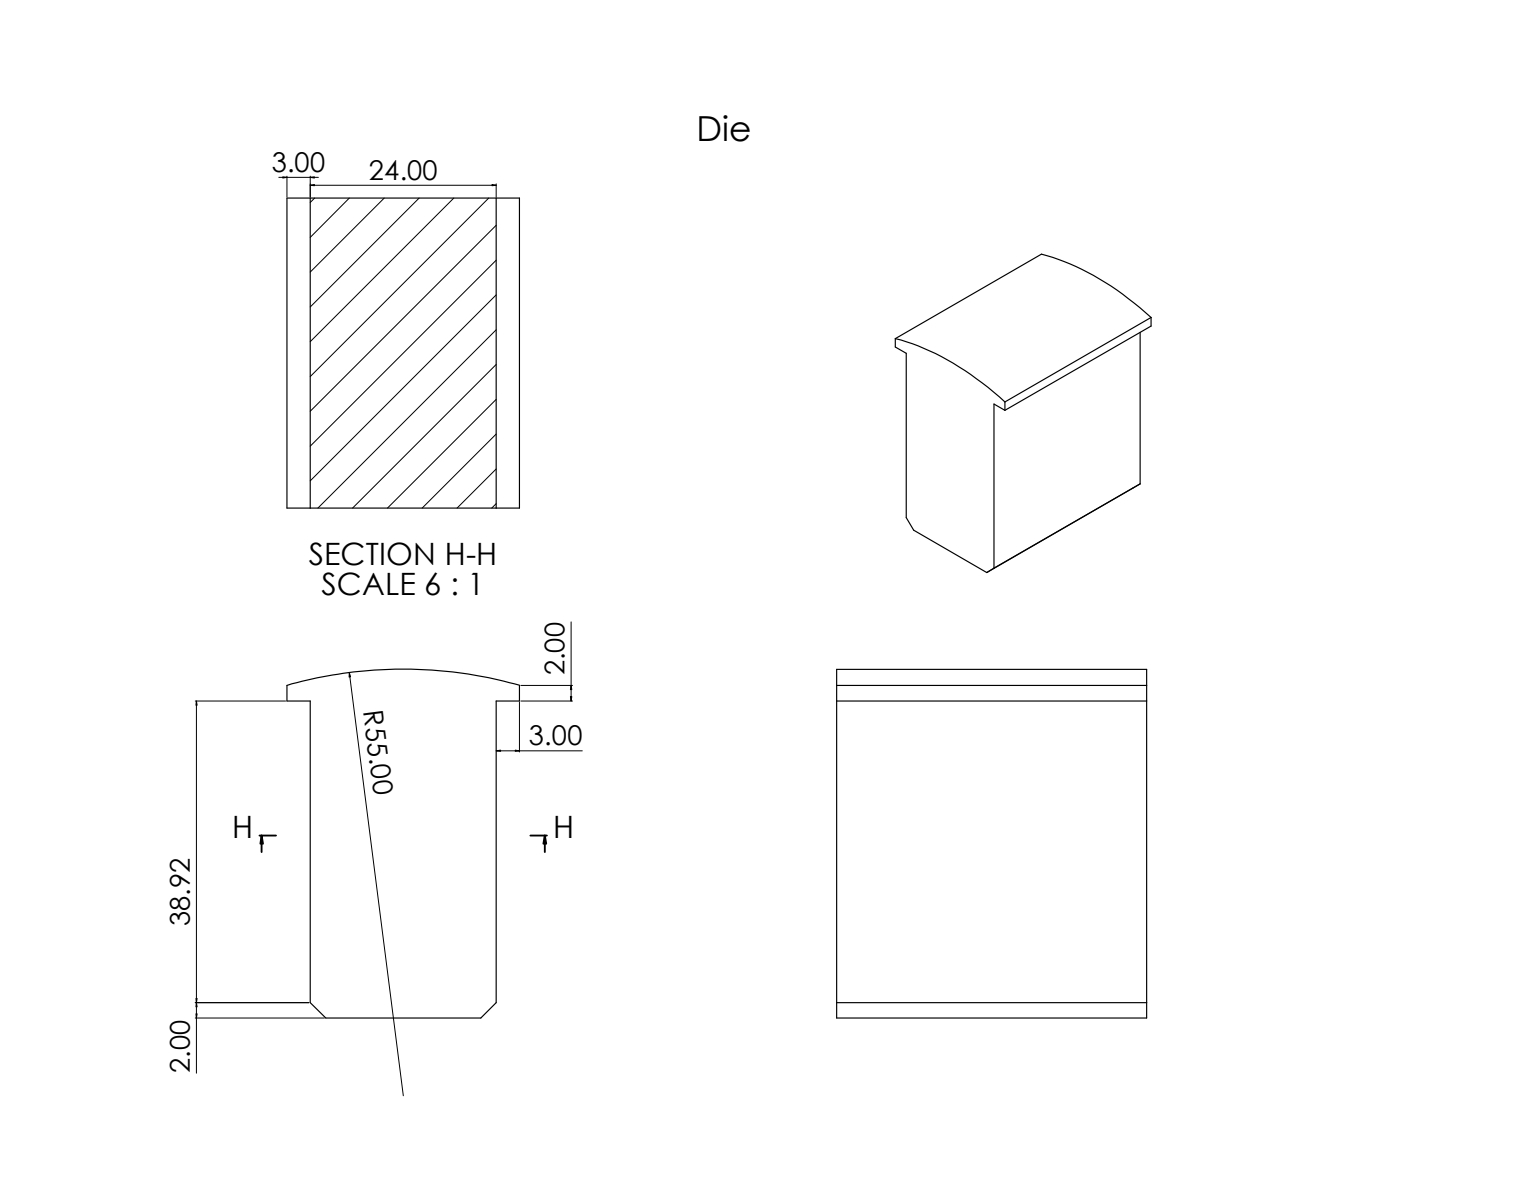
ISO-10303-21;
HEADER;
FILE_DESCRIPTION (('STEP AP214'),
    '1' );
FILE_NAME ('Die.step',
    '2026-10-25T19:19:31',
    ( '' ),
    ( '' ),
    'SwSTEP 2.0',
    'SolidWorks 2025',
    '' );
FILE_SCHEMA (( 'AUTOMOTIVE_DESIGN' ));
ENDSEC;

DATA;
#6=LINE ( 'NONE', #939, #4428 ) ;
#19=( NAMED_UNIT ( * ) SI_UNIT ( $, .STERADIAN. ) SOLID_ANGLE_UNIT ( ) );
#35=DIRECTION ( 'NONE',  ( 0.000000000000000000, -1.000000000000000000, 0.000000000000000000 ) ) ;
#40=APPLICATION_CONTEXT ( 'automotive_design' ) ;
#41=EDGE_CURVE ( 'NONE', #1178, #2811, #1439, .T. ) ;
#54=ORIENTED_EDGE ( 'NONE', *, *, #4887, .F. ) ;
#73=AXIS2_PLACEMENT_3D ( 'NONE', #3304, #3763, #5645 ) ;
#85=ORIENTED_EDGE ( 'NONE', *, *, #1081, .T. ) ;
#90=EDGE_CURVE ( 'NONE', #1861, #5383, #5968, .T. ) ;
#100=VECTOR ( 'NONE', #4962, 1000.000000000000000 ) ;
#127=EDGE_CURVE ( 'NONE', #4172, #3364, #4015, .T. ) ;
#185=EDGE_LOOP ( 'NONE', ( #533, #4724, #4763, #1601 ) ) ;
#202=AXIS2_PLACEMENT_3D ( 'NONE', #584, #4355, #522 ) ;
#232=ORIENTED_EDGE ( 'NONE', *, *, #1098, .F. ) ;
#233=FACE_OUTER_BOUND ( 'NONE', #1137, .T. ) ;
#242=ORIENTED_EDGE ( 'NONE', *, *, #2892, .F. ) ;
#249=MANIFOLD_SOLID_BREP ( 'Boss-Extrude4', #1653 ) ;
#255=LINE ( 'NONE', #729, #5225 ) ;
#274=DIRECTION ( 'NONE',  ( 0.000000000000000000, -1.000000000000000000, 0.000000000000000000 ) ) ;
#278=EDGE_LOOP ( 'NONE', ( #2591, #3538, #5453, #1395 ) ) ;
#289=DIRECTION ( 'NONE',  ( -0.000000000000000000, -0.000000000000000000, -1.000000000000000000 ) ) ;
#292=ADVANCED_FACE ( 'NONE', ( #988 ), #5742, .F. ) ;
#307=LINE ( 'NONE', #5608, #5057 ) ;
#321=DIRECTION ( 'NONE',  ( 1.000000000000000000, 8.673617379884026597E-16, -0.000000000000000000 ) ) ;
#329=PLANE ( 'NONE',  #2861 ) ;
#338=DIRECTION ( 'NONE',  ( -0.000000000000000000, -0.000000000000000000, -1.000000000000000000 ) ) ;
#350=EDGE_CURVE ( 'NONE', #4063, #382, #1866, .T. ) ;
#354=VERTEX_POINT ( 'NONE', #4776 ) ;
#382=VERTEX_POINT ( 'NONE', #5209 ) ;
#416=CARTESIAN_POINT ( 'NONE',  ( -15.00000000000000178, 52.91502622129182498, -20.00000000000000000 ) ) ;
#440=ORIENTED_EDGE ( 'NONE', *, *, #2522, .F. ) ;
#444=LINE ( 'NONE', #1490, #3945 ) ;
#451=CARTESIAN_POINT ( 'NONE',  ( -10.00000000000000178, 10.00000000000000178, -20.00000000000000000 ) ) ;
#475=AXIS2_PLACEMENT_3D ( 'NONE', #1088, #2025, #3550 ) ;
#489=ORIENTED_EDGE ( 'NONE', *, *, #127, .F. ) ;
#516=ORIENTED_EDGE ( 'NONE', *, *, #2045, .F. ) ;
#521=EDGE_CURVE ( 'NONE', #4734, #5727, #5427, .T. ) ;
#522=DIRECTION ( 'NONE',  ( -1.000000000000000000, 0.000000000000000000, 0.000000000000000000 ) ) ;
#533=ORIENTED_EDGE ( 'NONE', *, *, #4248, .T. ) ;
#546=ORIENTED_EDGE ( 'NONE', *, *, #4887, .T. ) ;
#584=CARTESIAN_POINT ( 'NONE',  ( 0.000000000000000000, 0.000000000000000000, 20.00000000000000000 ) ) ;
#636=ORIENTED_EDGE ( 'NONE', *, *, #827, .T. ) ;
#686=PLANE ( 'NONE',  #475 ) ;
#687=VECTOR ( 'NONE', #1691, 1000.000000000000000 ) ;
#707=VECTOR ( 'NONE', #2728, 1000.000000000000000 ) ;
#729=CARTESIAN_POINT ( 'NONE',  ( 9.999999999999998224, 9.999999999999998224, 20.00000000000000000 ) ) ;
#763=AXIS2_PLACEMENT_3D ( 'NONE', #4089, #6004, #1717 ) ;
#772=DIRECTION ( 'NONE',  ( -0.000000000000000000, 0.000000000000000000, 1.000000000000000000 ) ) ;
#773=LINE ( 'NONE', #3989, #1060 ) ;
#789=PLANE ( 'NONE',  #3246 ) ;
#793=EDGE_CURVE ( 'NONE', #354, #5786, #5696, .T. ) ;
#803=( GEOMETRIC_REPRESENTATION_CONTEXT ( 3 ) GLOBAL_UNCERTAINTY_ASSIGNED_CONTEXT ( ( #3805 ) ) GLOBAL_UNIT_ASSIGNED_CONTEXT ( ( #5845, #5678, #19 ) ) REPRESENTATION_CONTEXT ( 'NONE', 'WORKASPACE' ) );
#821=DIRECTION ( 'NONE',  ( 1.000000000000000000, -5.329070518200750605E-15, 0.000000000000000000 ) ) ;
#827=EDGE_CURVE ( 'NONE', #4272, #1861, #444, .T. ) ;
#870=VECTOR ( 'NONE', #3518, 1000.000000000000000 ) ;
#875=( GEOMETRIC_REPRESENTATION_CONTEXT ( 3 ) GLOBAL_UNCERTAINTY_ASSIGNED_CONTEXT ( ( #4308 ) ) GLOBAL_UNIT_ASSIGNED_CONTEXT ( ( #2245, #2215, #3729 ) ) REPRESENTATION_CONTEXT ( 'NONE', 'WORKASPACE' ) );
#898=SHAPE_REPRESENTATION_RELATIONSHIP ( 'NONE' , 'NONE' ,  #2176, #5744 ) ;
#930=LINE ( 'NONE', #958, #6029 ) ;
#939=CARTESIAN_POINT ( 'NONE',  ( -15.00000000000000178, 52.91502622129182498, 20.00000000000000000 ) ) ;
#945=VERTEX_POINT ( 'NONE', #1038 ) ;
#949=DIRECTION ( 'NONE',  ( -0.000000000000000000, -0.000000000000000000, -1.000000000000000000 ) ) ;
#958=CARTESIAN_POINT ( 'NONE',  ( 15.00000000000000178, 52.91502622129182498, 20.00000000000000000 ) ) ;
#970=PRODUCT ( 'Die', 'Die', '', ( #2146 ) ) ;
#988=FACE_OUTER_BOUND ( 'NONE', #1209, .T. ) ;
#992=VECTOR ( 'NONE', #1588, 1000.000000000000000 ) ;
#1022=DIRECTION ( 'NONE',  ( 1.000000000000000000, 0.000000000000000000, -0.000000000000000000 ) ) ;
#1038=CARTESIAN_POINT ( 'NONE',  ( -12.00000000000000000, 50.91502622129181788, 20.00000000000000000 ) ) ;
#1049=DIRECTION ( 'NONE',  ( -0.7071067811865469066, -0.7071067811865482389, 0.000000000000000000 ) ) ;
#1060=VECTOR ( 'NONE', #5434, 1000.000000000000000 ) ;
#1078=CARTESIAN_POINT ( 'NONE',  ( 12.00000000000000000, 50.91502622129181788, 20.00000000000000000 ) ) ;
#1081=EDGE_CURVE ( 'NONE', #1820, #382, #1825, .T. ) ;
#1088=CARTESIAN_POINT ( 'NONE',  ( 0.000000000000000000, 50.91502622129181788, 20.00000000000000000 ) ) ;
#1098=EDGE_CURVE ( 'NONE', #945, #1834, #307, .T. ) ;
#1110=DIRECTION ( 'NONE',  ( 0.000000000000000000, 1.000000000000000000, 0.000000000000000000 ) ) ;
#1122=ADVANCED_FACE ( 'NONE', ( #2775 ), #6053, .T. ) ;
#1131=ORIENTED_EDGE ( 'NONE', *, *, #5292, .T. ) ;
#1137=EDGE_LOOP ( 'NONE', ( #4292, #4354, #2571, #1131 ) ) ;
#1178=VERTEX_POINT ( 'NONE', #5278 ) ;
#1184=DIRECTION ( 'NONE',  ( -0.000000000000000000, 0.000000000000000000, 1.000000000000000000 ) ) ;
#1209=EDGE_LOOP ( 'NONE', ( #1696, #440, #232, #3423 ) ) ;
#1227=DIRECTION ( 'NONE',  ( 0.000000000000000000, -1.000000000000000000, 0.000000000000000000 ) ) ;
#1237=DIRECTION ( 'NONE',  ( -1.000000000000000000, 0.000000000000000000, 0.000000000000000000 ) ) ;
#1239=ORIENTED_EDGE ( 'NONE', *, *, #827, .F. ) ;
#1283=PLANE ( 'NONE',  #3222 ) ;
#1302=VERTEX_POINT ( 'NONE', #451 ) ;
#1335=VECTOR ( 'NONE', #338, 1000.000000000000000 ) ;
#1348=CIRCLE ( 'NONE', #2556, 55.00000000000001421 ) ;
#1387=PRODUCT_DEFINITION ( 'UNKNOWN', '', #4631, #2453 ) ;
#1392=DIRECTION ( 'NONE',  ( -0.000000000000000000, -0.000000000000000000, -1.000000000000000000 ) ) ;
#1395=ORIENTED_EDGE ( 'NONE', *, *, #3668, .T. ) ;
#1399=EDGE_CURVE ( 'NONE', #1672, #3029, #3458, .T. ) ;
#1405=CARTESIAN_POINT ( 'NONE',  ( 8.586443133426902668E-15, -8.586443133426886890E-15, 20.00000000000000000 ) ) ;
#1411=DIRECTION ( 'NONE',  ( -8.673617379884026597E-16, -1.000000000000000000, 0.000000000000000000 ) ) ;
#1424=CARTESIAN_POINT ( 'NONE',  ( -12.00000000000000000, 50.91502622129181788, -20.00000000000000000 ) ) ;
#1426=CARTESIAN_POINT ( 'NONE',  ( -11.99999999999999645, 12.00000000000000355, -20.00000000000000000 ) ) ;
#1439=LINE ( 'NONE', #2975, #4855 ) ;
#1490=CARTESIAN_POINT ( 'NONE',  ( 12.00000000000000000, 0.000000000000000000, -20.00000000000000000 ) ) ;
#1509=ORIENTED_EDGE ( 'NONE', *, *, #2047, .F. ) ;
#1525=DIRECTION ( 'NONE',  ( -0.000000000000000000, 0.000000000000000000, -1.000000000000000000 ) ) ;
#1530=ORIENTED_EDGE ( 'NONE', *, *, #2087, .T. ) ;
#1541=VECTOR ( 'NONE', #6048, 1000.000000000000000 ) ;
#1565=ADVANCED_FACE ( 'NONE', ( #5516 ), #329, .T. ) ;
#1571=VECTOR ( 'NONE', #5524, 1000.000000000000000 ) ;
#1583=FACE_OUTER_BOUND ( 'NONE', #278, .T. ) ;
#1588=DIRECTION ( 'NONE',  ( 8.673617379884026597E-16, -1.000000000000000000, 0.000000000000000000 ) ) ;
#1597=ORIENTED_EDGE ( 'NONE', *, *, #5103, .F. ) ;
#1601=ORIENTED_EDGE ( 'NONE', *, *, #2522, .T. ) ;
#1605=DIRECTION ( 'NONE',  ( 0.000000000000000000, -0.000000000000000000, -1.000000000000000000 ) ) ;
#1629=EDGE_CURVE ( 'NONE', #354, #1672, #6, .T. ) ;
#1651=CARTESIAN_POINT ( 'NONE',  ( -12.00000000000000000, 0.000000000000000000, -20.00000000000000000 ) ) ;
#1653=CLOSED_SHELL ( 'NONE', ( #3387, #2095, #2312, #292, #4074, #4285, #1565, #5408, #3225, #5043, #1122, #5390 ) ) ;
#1665=CARTESIAN_POINT ( 'NONE',  ( 9.999999999999998224, 9.999999999999998224, -20.00000000000000000 ) ) ;
#1672=VERTEX_POINT ( 'NONE', #416 ) ;
#1675=CARTESIAN_POINT ( 'NONE',  ( 8.586443133426902668E-15, -8.586443133426886890E-15, 20.00000000000000000 ) ) ;
#1691=DIRECTION ( 'NONE',  ( 0.000000000000000000, -1.000000000000000000, 0.000000000000000000 ) ) ;
#1692=FACE_OUTER_BOUND ( 'NONE', #4176, .T. ) ;
#1695=LINE ( 'NONE', #3172, #5157 ) ;
#1696=ORIENTED_EDGE ( 'NONE', *, *, #127, .T. ) ;
#1715=LINE ( 'NONE', #2497, #3224 ) ;
#1717=DIRECTION ( 'NONE',  ( -0.000000000000000000, 0.000000000000000000, -1.000000000000000000 ) ) ;
#1740=DIRECTION ( 'NONE',  ( 8.673617379884026597E-16, 1.000000000000000000, 0.000000000000000000 ) ) ;
#1758=DIRECTION ( 'NONE',  ( -0.000000000000000000, -0.000000000000000000, -1.000000000000000000 ) ) ;
#1820=VERTEX_POINT ( 'NONE', #3412 ) ;
#1825=LINE ( 'NONE', #4166, #1571 ) ;
#1834=VERTEX_POINT ( 'NONE', #4412 ) ;
#1861=VERTEX_POINT ( 'NONE', #3450 ) ;
#1866=LINE ( 'NONE', #1405, #5761 ) ;
#1945=CARTESIAN_POINT ( 'NONE',  ( -15.00000000000000000, 50.91502622129181788, 20.00000000000000000 ) ) ;
#1959=ORIENTED_EDGE ( 'NONE', *, *, #521, .T. ) ;
#1963=DIRECTION ( 'NONE',  ( -0.000000000000000000, -0.000000000000000000, -1.000000000000000000 ) ) ;
#1984=EDGE_CURVE ( 'NONE', #1302, #5383, #2197, .T. ) ;
#2025=DIRECTION ( 'NONE',  ( 0.000000000000000000, -1.000000000000000000, 0.000000000000000000 ) ) ;
#2032=CARTESIAN_POINT ( 'NONE',  ( -1.594625153350711036E-14, -1.594625153350706303E-14, 20.00000000000000000 ) ) ;
#2045=EDGE_CURVE ( 'NONE', #354, #4734, #1348, .T. ) ;
#2047=EDGE_CURVE ( 'NONE', #2811, #4272, #2698, .T. ) ;
#2087=EDGE_CURVE ( 'NONE', #3324, #4063, #3707, .T. ) ;
#2091=DIRECTION ( 'NONE',  ( -0.7071067811865469066, -0.7071067811865482389, 0.000000000000000000 ) ) ;
#2094=LINE ( 'NONE', #2032, #2125 ) ;
#2095=ADVANCED_FACE ( 'NONE', ( #3592 ), #789, .F. ) ;
#2110=SHAPE_DEFINITION_REPRESENTATION ( #3775, #2176 ) ;
#2125=VECTOR ( 'NONE', #5971, 1000.000000000000000 ) ;
#2146=PRODUCT_CONTEXT ( 'NONE', #40, 'mechanical' ) ;
#2156=ORIENTED_EDGE ( 'NONE', *, *, #5112, .T. ) ;
#2166=DIRECTION ( 'NONE',  ( 0.000000000000000000, -0.000000000000000000, -1.000000000000000000 ) ) ;
#2176=SHAPE_REPRESENTATION ( 'Die', ( #73 ), #875 ) ;
#2197=LINE ( 'NONE', #4625, #4943 ) ;
#2198=FACE_OUTER_BOUND ( 'NONE', #4368, .T. ) ;
#2215=( NAMED_UNIT ( * ) PLANE_ANGLE_UNIT ( ) SI_UNIT ( $, .RADIAN. ) );
#2245=( LENGTH_UNIT ( ) NAMED_UNIT ( * ) SI_UNIT ( .MILLI., .METRE. ) );
#2312=ADVANCED_FACE ( 'NONE', ( #233 ), #3139, .F. ) ;
#2313=ORIENTED_EDGE ( 'NONE', *, *, #5292, .F. ) ;
#2405=CARTESIAN_POINT ( 'NONE',  ( 15.00000000000000000, 50.91502622129181788, 20.00000000000000000 ) ) ;
#2453=PRODUCT_DEFINITION_CONTEXT ( 'detailed design', #2895, 'design' ) ;
#2463=CYLINDRICAL_SURFACE ( 'NONE', #202, 55.00000000000001421 ) ;
#2497=CARTESIAN_POINT ( 'NONE',  ( -1.594625153350711036E-14, -1.594625153350706303E-14, -20.00000000000000000 ) ) ;
#2522=EDGE_CURVE ( 'NONE', #1834, #3364, #3629, .T. ) ;
#2530=ORIENTED_EDGE ( 'NONE', *, *, #793, .T. ) ;
#2532=CARTESIAN_POINT ( 'NONE',  ( 14.99999999999995559, -1.301042606982600272E-14, 20.00000000000000000 ) ) ;
#2554=ORIENTED_EDGE ( 'NONE', *, *, #5378, .T. ) ;
#2556=AXIS2_PLACEMENT_3D ( 'NONE', #5101, #2166, #821 ) ;
#2559=DIRECTION ( 'NONE',  ( -0.000000000000000000, -0.000000000000000000, -1.000000000000000000 ) ) ;
#2571=ORIENTED_EDGE ( 'NONE', *, *, #3951, .F. ) ;
#2578=ORIENTED_EDGE ( 'NONE', *, *, #350, .F. ) ;
#2589=ORIENTED_EDGE ( 'NONE', *, *, #4893, .T. ) ;
#2591=ORIENTED_EDGE ( 'NONE', *, *, #1984, .T. ) ;
#2601=LINE ( 'NONE', #3962, #870 ) ;
#2618=EDGE_LOOP ( 'NONE', ( #516, #2530, #3475, #3498, #3096, #85, #2578, #3782, #54, #4075 ) ) ;
#2659=EDGE_LOOP ( 'NONE', ( #4184, #2313, #4641, #4438 ) ) ;
#2671=CARTESIAN_POINT ( 'NONE',  ( 0.000000000000000000, 0.000000000000000000, -20.00000000000000000 ) ) ;
#2686=LINE ( 'NONE', #4585, #1335 ) ;
#2698=LINE ( 'NONE', #4594, #5544 ) ;
#2699=PLANE ( 'NONE',  #763 ) ;
#2728=DIRECTION ( 'NONE',  ( -0.000000000000000000, -0.000000000000000000, -1.000000000000000000 ) ) ;
#2754=ORIENTED_EDGE ( 'NONE', *, *, #1984, .F. ) ;
#2775=FACE_OUTER_BOUND ( 'NONE', #2618, .T. ) ;
#2797=CARTESIAN_POINT ( 'NONE',  ( 12.00000000000000000, 12.00000000000000355, 20.00000000000000000 ) ) ;
#2811=VERTEX_POINT ( 'NONE', #6137 ) ;
#2814=ORIENTED_EDGE ( 'NONE', *, *, #5103, .T. ) ;
#2861=AXIS2_PLACEMENT_3D ( 'NONE', #1675, #3111, #5602 ) ;
#2890=DIRECTION ( 'NONE',  ( -0.7071067811865464625, 0.7071067811865486830, 0.000000000000000000 ) ) ;
#2892=EDGE_CURVE ( 'NONE', #3029, #4172, #1695, .T. ) ;
#2895=APPLICATION_CONTEXT ( 'automotive_design' ) ;
#2949=AXIS2_PLACEMENT_3D ( 'NONE', #3544, #4506, #4541 ) ;
#2975=CARTESIAN_POINT ( 'NONE',  ( 14.99999999999995559, -1.301042606982600272E-14, -20.00000000000000000 ) ) ;
#2992=EDGE_LOOP ( 'NONE', ( #1597, #5836, #5687, #3359 ) ) ;
#3029=VERTEX_POINT ( 'NONE', #5195 ) ;
#3076=DIRECTION ( 'NONE',  ( 1.000000000000000000, 0.000000000000000000, 0.000000000000000000 ) ) ;
#3093=CARTESIAN_POINT ( 'NONE',  ( 8.586443133426902668E-15, -8.586443133426886890E-15, -20.00000000000000000 ) ) ;
#3096=ORIENTED_EDGE ( 'NONE', *, *, #4794, .T. ) ;
#3111=DIRECTION ( 'NONE',  ( 0.7071067811865482389, -0.7071067811865469066, 0.000000000000000000 ) ) ;
#3115=CARTESIAN_POINT ( 'NONE',  ( 12.00000000000000000, 50.91502622129181788, 20.00000000000000000 ) ) ;
#3139=PLANE ( 'NONE',  #2949 ) ;
#3140=ORIENTED_EDGE ( 'NONE', *, *, #4248, .F. ) ;
#3156=ORIENTED_EDGE ( 'NONE', *, *, #5799, .F. ) ;
#3158=STYLED_ITEM('',(#6170),#249);
#3172=CARTESIAN_POINT ( 'NONE',  ( -0.000000000000000000, 50.91502622129181788, -20.00000000000000000 ) ) ;
#3201=ORIENTED_EDGE ( 'NONE', *, *, #350, .T. ) ;
#3222=AXIS2_PLACEMENT_3D ( 'NONE', #5091, #5060, #1740 ) ;
#3224=VECTOR ( 'NONE', #5298, 1000.000000000000000 ) ;
#3225=ADVANCED_FACE ( 'NONE', ( #5963 ), #686, .T. ) ;
#3246=AXIS2_PLACEMENT_3D ( 'NONE', #4088, #321, #6003 ) ;
#3291=ORIENTED_EDGE ( 'NONE', *, *, #2047, .T. ) ;
#3304=CARTESIAN_POINT ( 'NONE',  ( 0.000000000000000000, 0.000000000000000000, 0.000000000000000000 ) ) ;
#3324=VERTEX_POINT ( 'NONE', #3115 ) ;
#3331=LINE ( 'NONE', #2405, #5825 ) ;
#3359=ORIENTED_EDGE ( 'NONE', *, *, #5799, .T. ) ;
#3364=VERTEX_POINT ( 'NONE', #1426 ) ;
#3367=CARTESIAN_POINT ( 'NONE',  ( -12.00000000000000000, 0.000000000000000000, 20.00000000000000000 ) ) ;
#3387=ADVANCED_FACE ( 'NONE', ( #4289 ), #2463, .T. ) ;
#3412=CARTESIAN_POINT ( 'NONE',  ( -10.00000000000000178, 10.00000000000000178, 20.00000000000000000 ) ) ;
#3423=ORIENTED_EDGE ( 'NONE', *, *, #5072, .T. ) ;
#3450=CARTESIAN_POINT ( 'NONE',  ( 12.00000000000000000, 12.00000000000000355, -20.00000000000000000 ) ) ;
#3458=LINE ( 'NONE', #3917, #992 ) ;
#3475=ORIENTED_EDGE ( 'NONE', *, *, #3951, .T. ) ;
#3481=DIRECTION ( 'NONE',  ( 0.000000000000000000, -0.000000000000000000, 1.000000000000000000 ) ) ;
#3498=ORIENTED_EDGE ( 'NONE', *, *, #1098, .T. ) ;
#3500=EDGE_CURVE ( 'NONE', #3324, #4272, #4898, .T. ) ;
#3518=DIRECTION ( 'NONE',  ( -1.000000000000000000, 0.000000000000000000, 0.000000000000000000 ) ) ;
#3538=ORIENTED_EDGE ( 'NONE', *, *, #5378, .F. ) ;
#3544=CARTESIAN_POINT ( 'NONE',  ( 0.000000000000000000, 50.91502622129181788, 20.00000000000000000 ) ) ;
#3550=DIRECTION ( 'NONE',  ( 0.000000000000000000, -0.000000000000000000, -1.000000000000000000 ) ) ;
#3552=VECTOR ( 'NONE', #4258, 1000.000000000000000 ) ;
#3563=VECTOR ( 'NONE', #1963, 1000.000000000000000 ) ;
#3592=FACE_OUTER_BOUND ( 'NONE', #2659, .T. ) ;
#3593=PLANE ( 'NONE',  #4824 ) ;
#3595=DIRECTION ( 'NONE',  ( 1.000000000000000000, 0.000000000000000000, 0.000000000000000000 ) ) ;
#3611=ORIENTED_EDGE ( 'NONE', *, *, #1399, .F. ) ;
#3619=AXIS2_PLACEMENT_3D ( 'NONE', #4316, #6102, #2890 ) ;
#3629=LINE ( 'NONE', #5547, #707 ) ;
#3668=EDGE_CURVE ( 'NONE', #1820, #1302, #6111, .T. ) ;
#3707=LINE ( 'NONE', #5978, #687 ) ;
#3709=AXIS2_PLACEMENT_3D ( 'NONE', #4295, #1605, #4228 ) ;
#3729=( NAMED_UNIT ( * ) SI_UNIT ( $, .STERADIAN. ) SOLID_ANGLE_UNIT ( ) );
#3735=EDGE_LOOP ( 'NONE', ( #4808, #4256, #3201, #2554 ) ) ;
#3760=CARTESIAN_POINT ( 'NONE',  ( -15.00000000000000000, 50.91502622129181788, 20.00000000000000000 ) ) ;
#3763=DIRECTION ( 'NONE',  ( 0.000000000000000000, 0.000000000000000000, 1.000000000000000000 ) ) ;
#3775=PRODUCT_DEFINITION_SHAPE ( 'NONE', 'NONE',  #1387 ) ;
#3782=ORIENTED_EDGE ( 'NONE', *, *, #2087, .F. ) ;
#3805=UNCERTAINTY_MEASURE_WITH_UNIT (LENGTH_MEASURE( 1.000000000000000082E-05 ), #5845, 'distance_accuracy_value', 'NONE');
#3808=EDGE_LOOP ( 'NONE', ( #1509, #5655, #546, #5484 ) ) ;
#3849=FACE_OUTER_BOUND ( 'NONE', #185, .T. ) ;
#3901=ORIENTED_EDGE ( 'NONE', *, *, #41, .F. ) ;
#3917=CARTESIAN_POINT ( 'NONE',  ( -14.99999999999995559, -1.301042606982600272E-14, -20.00000000000000000 ) ) ;
#3944=CARTESIAN_POINT ( 'NONE',  ( 12.00000000000000000, 50.91502622129181788, -20.00000000000000000 ) ) ;
#3945=VECTOR ( 'NONE', #35, 1000.000000000000000 ) ;
#3951=EDGE_CURVE ( 'NONE', #5786, #945, #4134, .T. ) ;
#3962=CARTESIAN_POINT ( 'NONE',  ( 0.000000000000000000, 50.91502622129181788, 20.00000000000000000 ) ) ;
#3977=ORIENTED_EDGE ( 'NONE', *, *, #90, .T. ) ;
#3989=CARTESIAN_POINT ( 'NONE',  ( 12.00000000000000000, 12.00000000000000355, 20.00000000000000000 ) ) ;
#4015=LINE ( 'NONE', #1651, #4234 ) ;
#4063=VERTEX_POINT ( 'NONE', #2797 ) ;
#4074=ADVANCED_FACE ( 'NONE', ( #3849 ), #4695, .F. ) ;
#4075=ORIENTED_EDGE ( 'NONE', *, *, #521, .F. ) ;
#4088=CARTESIAN_POINT ( 'NONE',  ( -14.99999999999995559, -1.301042606982600272E-14, 20.00000000000000000 ) ) ;
#4089=CARTESIAN_POINT ( 'NONE',  ( 12.00000000000000000, 0.000000000000000000, 20.00000000000000000 ) ) ;
#4134=LINE ( 'NONE', #4162, #1541 ) ;
#4162=CARTESIAN_POINT ( 'NONE',  ( 0.000000000000000000, 50.91502622129181788, 20.00000000000000000 ) ) ;
#4166=CARTESIAN_POINT ( 'NONE',  ( 0.000000000000000000, 9.999999999999998224, 20.00000000000000000 ) ) ;
#4172=VERTEX_POINT ( 'NONE', #1424 ) ;
#4176=EDGE_LOOP ( 'NONE', ( #2814, #5535, #3291, #636, #3977, #2754, #3140, #489, #242, #3611 ) ) ;
#4184=ORIENTED_EDGE ( 'NONE', *, *, #1399, .T. ) ;
#4228=DIRECTION ( 'NONE',  ( 1.000000000000000000, -5.329070518200750605E-15, 0.000000000000000000 ) ) ;
#4234=VECTOR ( 'NONE', #274, 1000.000000000000000 ) ;
#4238=DIRECTION ( 'NONE',  ( -0.000000000000000000, -0.000000000000000000, -1.000000000000000000 ) ) ;
#4248=EDGE_CURVE ( 'NONE', #3364, #1302, #1715, .T. ) ;
#4256=ORIENTED_EDGE ( 'NONE', *, *, #4893, .F. ) ;
#4258=DIRECTION ( 'NONE',  ( 8.673617379884026597E-16, -1.000000000000000000, 0.000000000000000000 ) ) ;
#4272=VERTEX_POINT ( 'NONE', #3944 ) ;
#4285=ADVANCED_FACE ( 'NONE', ( #1583 ), #5829, .F. ) ;
#4289=FACE_OUTER_BOUND ( 'NONE', #2992, .T. ) ;
#4292=ORIENTED_EDGE ( 'NONE', *, *, #2892, .T. ) ;
#4295=CARTESIAN_POINT ( 'NONE',  ( 0.000000000000000000, 0.000000000000000000, -20.00000000000000000 ) ) ;
#4308=UNCERTAINTY_MEASURE_WITH_UNIT (LENGTH_MEASURE( 1.000000000000000082E-05 ), #2245, 'distance_accuracy_value', 'NONE');
#4315=CIRCLE ( 'NONE', #3709, 55.00000000000001421 ) ;
#4316=CARTESIAN_POINT ( 'NONE',  ( -1.594625153350711036E-14, -1.594625153350706303E-14, 20.00000000000000000 ) ) ;
#4354=ORIENTED_EDGE ( 'NONE', *, *, #5072, .F. ) ;
#4355=DIRECTION ( 'NONE',  ( -0.000000000000000000, -0.000000000000000000, -1.000000000000000000 ) ) ;
#4368=EDGE_LOOP ( 'NONE', ( #1239, #5607, #1530, #2589 ) ) ;
#4412=CARTESIAN_POINT ( 'NONE',  ( -11.99999999999999645, 12.00000000000000355, 20.00000000000000000 ) ) ;
#4428=VECTOR ( 'NONE', #1392, 1000.000000000000000 ) ;
#4438=ORIENTED_EDGE ( 'NONE', *, *, #1629, .T. ) ;
#4506=DIRECTION ( 'NONE',  ( 0.000000000000000000, 1.000000000000000000, 0.000000000000000000 ) ) ;
#4541=DIRECTION ( 'NONE',  ( 0.000000000000000000, -0.000000000000000000, 1.000000000000000000 ) ) ;
#4551=DIRECTION ( 'NONE',  ( 1.000000000000000000, 0.000000000000000000, 0.000000000000000000 ) ) ;
#4559=AXIS2_PLACEMENT_3D ( 'NONE', #3367, #1022, #1525 ) ;
#4565=CARTESIAN_POINT ( 'NONE',  ( 15.00000000000000000, 50.91502622129181788, 20.00000000000000000 ) ) ;
#4585=CARTESIAN_POINT ( 'NONE',  ( -12.00000000000000000, 50.91502622129181788, 20.00000000000000000 ) ) ;
#4594=CARTESIAN_POINT ( 'NONE',  ( 0.000000000000000000, 50.91502622129181788, -20.00000000000000000 ) ) ;
#4625=CARTESIAN_POINT ( 'NONE',  ( -0.000000000000000000, 9.999999999999998224, -20.00000000000000000 ) ) ;
#4631=PRODUCT_DEFINITION_FORMATION_WITH_SPECIFIED_SOURCE ( 'ANY', '', #970, .NOT_KNOWN. ) ;
#4641=ORIENTED_EDGE ( 'NONE', *, *, #793, .F. ) ;
#4658=DIRECTION ( 'NONE',  ( 1.000000000000000000, 0.000000000000000000, 0.000000000000000000 ) ) ;
#4695=PLANE ( 'NONE',  #3619 ) ;
#4724=ORIENTED_EDGE ( 'NONE', *, *, #3668, .F. ) ;
#4726=AXIS2_PLACEMENT_3D ( 'NONE', #5328, #1110, #3481 ) ;
#4734=VERTEX_POINT ( 'NONE', #5908 ) ;
#4763=ORIENTED_EDGE ( 'NONE', *, *, #4794, .F. ) ;
#4776=CARTESIAN_POINT ( 'NONE',  ( -15.00000000000000178, 52.91502622129182498, 20.00000000000000000 ) ) ;
#4794=EDGE_CURVE ( 'NONE', #1834, #1820, #2094, .T. ) ;
#4806=CARTESIAN_POINT ( 'NONE',  ( -10.00000000000000178, 10.00000000000000178, 20.00000000000000000 ) ) ;
#4808=ORIENTED_EDGE ( 'NONE', *, *, #90, .F. ) ;
#4824=AXIS2_PLACEMENT_3D ( 'NONE', #2671, #1184, #3076 ) ;
#4855=VECTOR ( 'NONE', #1411, 1000.000000000000000 ) ;
#4868=AXIS2_PLACEMENT_3D ( 'NONE', #5027, #772, #4551 ) ;
#4887=EDGE_CURVE ( 'NONE', #5727, #3324, #2601, .T. ) ;
#4893=EDGE_CURVE ( 'NONE', #4063, #1861, #773, .T. ) ;
#4898=LINE ( 'NONE', #1078, #5662 ) ;
#4943=VECTOR ( 'NONE', #4658, 1000.000000000000000 ) ;
#4962=DIRECTION ( 'NONE',  ( -8.673617379884026597E-16, -1.000000000000000000, 0.000000000000000000 ) ) ;
#5027=CARTESIAN_POINT ( 'NONE',  ( 0.000000000000000000, 0.000000000000000000, 20.00000000000000000 ) ) ;
#5043=ADVANCED_FACE ( 'NONE', ( #5116 ), #1283, .T. ) ;
#5057=VECTOR ( 'NONE', #1227, 1000.000000000000000 ) ;
#5060=DIRECTION ( 'NONE',  ( 1.000000000000000000, -8.673617379884026597E-16, 0.000000000000000000 ) ) ;
#5072=EDGE_CURVE ( 'NONE', #945, #4172, #2686, .T. ) ;
#5091=CARTESIAN_POINT ( 'NONE',  ( 14.99999999999995559, -1.301042606982600272E-14, 20.00000000000000000 ) ) ;
#5101=CARTESIAN_POINT ( 'NONE',  ( 0.000000000000000000, 0.000000000000000000, 20.00000000000000000 ) ) ;
#5103=EDGE_CURVE ( 'NONE', #1672, #1178, #4315, .T. ) ;
#5112=EDGE_CURVE ( 'NONE', #5727, #2811, #3331, .T. ) ;
#5116=FACE_OUTER_BOUND ( 'NONE', #5710, .T. ) ;
#5157=VECTOR ( 'NONE', #3595, 1000.000000000000000 ) ;
#5195=CARTESIAN_POINT ( 'NONE',  ( -15.00000000000000000, 50.91502622129181788, -20.00000000000000000 ) ) ;
#5209=CARTESIAN_POINT ( 'NONE',  ( 9.999999999999998224, 9.999999999999998224, 20.00000000000000000 ) ) ;
#5225=VECTOR ( 'NONE', #289, 1000.000000000000000 ) ;
#5235=CARTESIAN_POINT ( 'NONE',  ( -14.99999999999995559, -1.301042606982600272E-14, 20.00000000000000000 ) ) ;
#5278=CARTESIAN_POINT ( 'NONE',  ( 15.00000000000000178, 52.91502622129182498, -20.00000000000000000 ) ) ;
#5292=EDGE_CURVE ( 'NONE', #5786, #3029, #5888, .T. ) ;
#5298=DIRECTION ( 'NONE',  ( 0.7071067811865464625, -0.7071067811865486830, 0.000000000000000000 ) ) ;
#5328=CARTESIAN_POINT ( 'NONE',  ( 0.000000000000000000, 9.999999999999998224, 20.00000000000000000 ) ) ;
#5378=EDGE_CURVE ( 'NONE', #382, #5383, #255, .T. ) ;
#5383=VERTEX_POINT ( 'NONE', #1665 ) ;
#5390=ADVANCED_FACE ( 'NONE', ( #1692 ), #3593, .F. ) ;
#5408=ADVANCED_FACE ( 'NONE', ( #2198 ), #2699, .T. ) ;
#5427=LINE ( 'NONE', #2532, #100 ) ;
#5434=DIRECTION ( 'NONE',  ( -0.000000000000000000, -0.000000000000000000, -1.000000000000000000 ) ) ;
#5453=ORIENTED_EDGE ( 'NONE', *, *, #1081, .F. ) ;
#5484=ORIENTED_EDGE ( 'NONE', *, *, #3500, .T. ) ;
#5516=FACE_OUTER_BOUND ( 'NONE', #3735, .T. ) ;
#5520=VECTOR ( 'NONE', #1758, 1000.000000000000000 ) ;
#5524=DIRECTION ( 'NONE',  ( 1.000000000000000000, 0.000000000000000000, 0.000000000000000000 ) ) ;
#5535=ORIENTED_EDGE ( 'NONE', *, *, #41, .T. ) ;
#5544=VECTOR ( 'NONE', #1237, 1000.000000000000000 ) ;
#5547=CARTESIAN_POINT ( 'NONE',  ( -11.99999999999999645, 12.00000000000000355, 20.00000000000000000 ) ) ;
#5602=DIRECTION ( 'NONE',  ( 0.7071067811865469066, 0.7071067811865482389, 0.000000000000000000 ) ) ;
#5607=ORIENTED_EDGE ( 'NONE', *, *, #3500, .F. ) ;
#5608=CARTESIAN_POINT ( 'NONE',  ( -12.00000000000000000, 0.000000000000000000, 20.00000000000000000 ) ) ;
#5639=VECTOR ( 'NONE', #2091, 999.9999999999998863 ) ;
#5645=DIRECTION ( 'NONE',  ( 1.000000000000000000, 0.000000000000000000, 0.000000000000000000 ) ) ;
#5655=ORIENTED_EDGE ( 'NONE', *, *, #5112, .F. ) ;
#5662=VECTOR ( 'NONE', #2559, 1000.000000000000000 ) ;
#5678=( NAMED_UNIT ( * ) PLANE_ANGLE_UNIT ( ) SI_UNIT ( $, .RADIAN. ) );
#5687=ORIENTED_EDGE ( 'NONE', *, *, #2045, .T. ) ;
#5696=LINE ( 'NONE', #5235, #3552 ) ;
#5710=EDGE_LOOP ( 'NONE', ( #3901, #3156, #1959, #2156 ) ) ;
#5727=VERTEX_POINT ( 'NONE', #4565 ) ;
#5742=PLANE ( 'NONE',  #4559 ) ;
#5744=ADVANCED_BREP_SHAPE_REPRESENTATION ( '', ( #249, #73 ), #875 ) ;
#5761=VECTOR ( 'NONE', #1049, 999.9999999999998863 ) ;
#5786=VERTEX_POINT ( 'NONE', #1945 ) ;
#5799=EDGE_CURVE ( 'NONE', #4734, #1178, #930, .T. ) ;
#5825=VECTOR ( 'NONE', #949, 1000.000000000000000 ) ;
#5829=PLANE ( 'NONE',  #4726 ) ;
#5836=ORIENTED_EDGE ( 'NONE', *, *, #1629, .F. ) ;
#5845=( LENGTH_UNIT ( ) NAMED_UNIT ( * ) SI_UNIT ( .MILLI., .METRE. ) );
#5857=MECHANICAL_DESIGN_GEOMETRIC_PRESENTATION_REPRESENTATION('',(#3158),#803);
#5888=LINE ( 'NONE', #3760, #5520 ) ;
#5908=CARTESIAN_POINT ( 'NONE',  ( 15.00000000000000178, 52.91502622129182498, 20.00000000000000000 ) ) ;
#5963=FACE_OUTER_BOUND ( 'NONE', #3808, .T. ) ;
#5968=LINE ( 'NONE', #3093, #5639 ) ;
#5971=DIRECTION ( 'NONE',  ( 0.7071067811865464625, -0.7071067811865486830, 0.000000000000000000 ) ) ;
#5978=CARTESIAN_POINT ( 'NONE',  ( 12.00000000000000000, 0.000000000000000000, 20.00000000000000000 ) ) ;
#6003=DIRECTION ( 'NONE',  ( -8.673617379884026597E-16, 1.000000000000000000, 0.000000000000000000 ) ) ;
#6004=DIRECTION ( 'NONE',  ( 1.000000000000000000, 0.000000000000000000, -0.000000000000000000 ) ) ;
#6029=VECTOR ( 'NONE', #4238, 1000.000000000000000 ) ;
#6048=DIRECTION ( 'NONE',  ( 1.000000000000000000, 0.000000000000000000, 0.000000000000000000 ) ) ;
#6053=PLANE ( 'NONE',  #4868 ) ;
#6102=DIRECTION ( 'NONE',  ( 0.7071067811865486830, 0.7071067811865464625, -0.000000000000000000 ) ) ;
#6111=LINE ( 'NONE', #4806, #3563 ) ;
#6137=CARTESIAN_POINT ( 'NONE',  ( 15.00000000000000000, 50.91502622129181788, -20.00000000000000000 ) ) ;
#6164=COLOUR_RGB('Light Blue',0.38,0.62,0.78);
#6165=FILL_AREA_STYLE_COLOUR('',#6164);
#6166=FILL_AREA_STYLE('',(#6165));
#6167=SURFACE_STYLE_FILL_AREA(#6166);
#6168=SURFACE_SIDE_STYLE('',(#6167));
#6169=SURFACE_STYLE_USAGE(.BOTH.,#6168);
#6170=PRESENTATION_STYLE_ASSIGNMENT((#6169));
ENDSEC;
END-ISO-10303-21;
